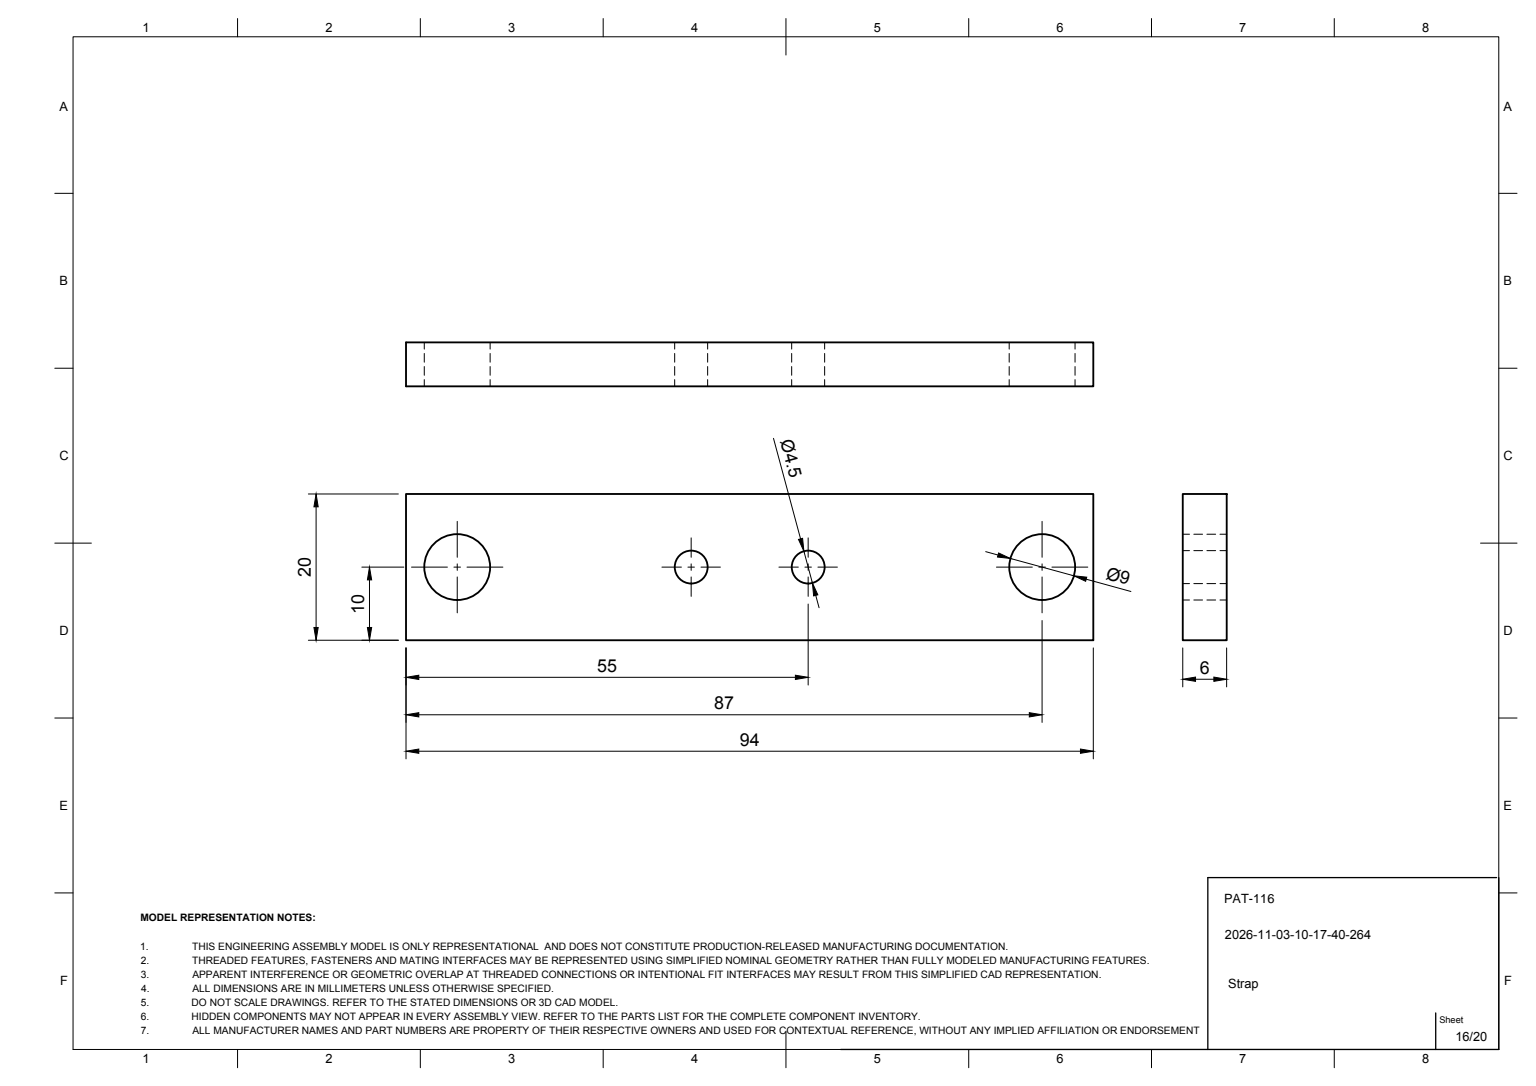
ISO-10303-21;
HEADER;
/* Generated by software containing ST-Developer
 * from STEP Tools, Inc. (www.steptools.com) 
 */

FILE_DESCRIPTION(
/* description */ ('V-block with clamp strap'),
/* implementation_level */ '2;1');

FILE_NAME(
/* name */ 'Strap.step',
/* time_stamp */ '2026-10-27T10:50:53-07:00',
/* author */ (''),
/* organization */ (''),
/* preprocessor_version */ 'ST-DEVELOPER v20.2',
/* originating_system */ 'Autodesk Translation Framework v15.17.0.0',
/* authorisation */ '');

FILE_SCHEMA (('AUTOMOTIVE_DESIGN { 1 0 10303 214 3 1 1 }'));
ENDSEC;

DATA;
#10=MECHANICAL_DESIGN_GEOMETRIC_PRESENTATION_REPRESENTATION('',(#279),#7344);
#237=SHAPE_REPRESENTATION_RELATIONSHIP('SRR','None',#7456,#258);
#258=ADVANCED_BREP_SHAPE_REPRESENTATION('',(#298),#7335);
#279=STYLED_ITEM('',(#7645),#298);
#298=MANIFOLD_SOLID_BREP('Body1',#4163);
#361=FACE_BOUND('',#1047,.T.);
#362=FACE_BOUND('',#1048,.T.);
#363=FACE_BOUND('',#1049,.T.);
#364=FACE_BOUND('',#1050,.T.);
#365=FACE_BOUND('',#1052,.T.);
#366=FACE_BOUND('',#1053,.T.);
#367=FACE_BOUND('',#1054,.T.);
#368=FACE_BOUND('',#1055,.T.);
#470=CIRCLE('',#4723,0.225);
#471=CIRCLE('',#4724,0.225);
#472=CIRCLE('',#4726,0.225);
#473=CIRCLE('',#4727,0.225);
#474=CIRCLE('',#4729,0.449999999999999);
#475=CIRCLE('',#4730,0.449999999999999);
#476=CIRCLE('',#4732,0.449999999999999);
#477=CIRCLE('',#4733,0.449999999999999);
#547=CYLINDRICAL_SURFACE('',#4722,0.225);
#548=CYLINDRICAL_SURFACE('',#4725,0.225);
#549=CYLINDRICAL_SURFACE('',#4728,0.449999999999999);
#550=CYLINDRICAL_SURFACE('',#4731,0.449999999999999);
#742=FACE_OUTER_BOUND('',#1038,.T.);
#743=FACE_OUTER_BOUND('',#1039,.T.);
#744=FACE_OUTER_BOUND('',#1040,.T.);
#745=FACE_OUTER_BOUND('',#1041,.T.);
#746=FACE_OUTER_BOUND('',#1042,.T.);
#747=FACE_OUTER_BOUND('',#1043,.T.);
#748=FACE_OUTER_BOUND('',#1044,.T.);
#749=FACE_OUTER_BOUND('',#1045,.T.);
#750=FACE_OUTER_BOUND('',#1046,.T.);
#751=FACE_OUTER_BOUND('',#1051,.T.);
#1038=EDGE_LOOP('',(#3516,#3517,#3518,#3519));
#1039=EDGE_LOOP('',(#3520,#3521,#3522,#3523));
#1040=EDGE_LOOP('',(#3524,#3525,#3526,#3527));
#1041=EDGE_LOOP('',(#3528,#3529,#3530,#3531));
#1042=EDGE_LOOP('',(#3532,#3533,#3534,#3535));
#1043=EDGE_LOOP('',(#3536,#3537,#3538,#3539));
#1044=EDGE_LOOP('',(#3540,#3541,#3542,#3543));
#1045=EDGE_LOOP('',(#3544,#3545,#3546,#3547));
#1046=EDGE_LOOP('',(#3548,#3549,#3550,#3551));
#1047=EDGE_LOOP('',(#3552));
#1048=EDGE_LOOP('',(#3553));
#1049=EDGE_LOOP('',(#3554));
#1050=EDGE_LOOP('',(#3555));
#1051=EDGE_LOOP('',(#3556,#3557,#3558,#3559));
#1052=EDGE_LOOP('',(#3560));
#1053=EDGE_LOOP('',(#3561));
#1054=EDGE_LOOP('',(#3562));
#1055=EDGE_LOOP('',(#3563));
#1413=LINE('',#7002,#1778);
#1414=LINE('',#7008,#1779);
#1415=LINE('',#7014,#1780);
#1416=LINE('',#7020,#1781);
#1417=LINE('',#7025,#1782);
#1418=LINE('',#7027,#1783);
#1419=LINE('',#7029,#1784);
#1420=LINE('',#7030,#1785);
#1421=LINE('',#7033,#1786);
#1422=LINE('',#7035,#1787);
#1423=LINE('',#7036,#1788);
#1424=LINE('',#7039,#1789);
#1425=LINE('',#7041,#1790);
#1426=LINE('',#7042,#1791);
#1427=LINE('',#7044,#1792);
#1428=LINE('',#7045,#1793);
#1778=VECTOR('',#5783,0.225);
#1779=VECTOR('',#5790,0.225);
#1780=VECTOR('',#5797,0.449999999999999);
#1781=VECTOR('',#5804,0.449999999999999);
#1782=VECTOR('',#5809,1.);
#1783=VECTOR('',#5810,1.);
#1784=VECTOR('',#5811,1.);
#1785=VECTOR('',#5812,1.);
#1786=VECTOR('',#5815,1.);
#1787=VECTOR('',#5816,1.);
#1788=VECTOR('',#5817,1.);
#1789=VECTOR('',#5820,1.);
#1790=VECTOR('',#5821,1.);
#1791=VECTOR('',#5822,1.);
#1792=VECTOR('',#5825,1.);
#1793=VECTOR('',#5826,1.);
#2101=VERTEX_POINT('',#6999);
#2102=VERTEX_POINT('',#7001);
#2103=VERTEX_POINT('',#7005);
#2104=VERTEX_POINT('',#7007);
#2105=VERTEX_POINT('',#7011);
#2106=VERTEX_POINT('',#7013);
#2107=VERTEX_POINT('',#7017);
#2108=VERTEX_POINT('',#7019);
#2109=VERTEX_POINT('',#7023);
#2110=VERTEX_POINT('',#7024);
#2111=VERTEX_POINT('',#7026);
#2112=VERTEX_POINT('',#7028);
#2113=VERTEX_POINT('',#7032);
#2114=VERTEX_POINT('',#7034);
#2115=VERTEX_POINT('',#7038);
#2116=VERTEX_POINT('',#7040);
#2584=EDGE_CURVE('',#2101,#2101,#470,.T.);
#2585=EDGE_CURVE('',#2101,#2102,#1413,.T.);
#2586=EDGE_CURVE('',#2102,#2102,#471,.T.);
#2587=EDGE_CURVE('',#2103,#2103,#472,.T.);
#2588=EDGE_CURVE('',#2103,#2104,#1414,.T.);
#2589=EDGE_CURVE('',#2104,#2104,#473,.T.);
#2590=EDGE_CURVE('',#2105,#2105,#474,.T.);
#2591=EDGE_CURVE('',#2105,#2106,#1415,.T.);
#2592=EDGE_CURVE('',#2106,#2106,#475,.T.);
#2593=EDGE_CURVE('',#2107,#2107,#476,.T.);
#2594=EDGE_CURVE('',#2107,#2108,#1416,.T.);
#2595=EDGE_CURVE('',#2108,#2108,#477,.T.);
#2596=EDGE_CURVE('',#2109,#2110,#1417,.T.);
#2597=EDGE_CURVE('',#2110,#2111,#1418,.T.);
#2598=EDGE_CURVE('',#2112,#2111,#1419,.T.);
#2599=EDGE_CURVE('',#2109,#2112,#1420,.T.);
#2600=EDGE_CURVE('',#2113,#2109,#1421,.T.);
#2601=EDGE_CURVE('',#2114,#2112,#1422,.T.);
#2602=EDGE_CURVE('',#2113,#2114,#1423,.T.);
#2603=EDGE_CURVE('',#2115,#2113,#1424,.T.);
#2604=EDGE_CURVE('',#2116,#2114,#1425,.T.);
#2605=EDGE_CURVE('',#2115,#2116,#1426,.T.);
#2606=EDGE_CURVE('',#2110,#2115,#1427,.T.);
#2607=EDGE_CURVE('',#2111,#2116,#1428,.T.);
#3516=ORIENTED_EDGE('',*,*,#2584,.F.);
#3517=ORIENTED_EDGE('',*,*,#2585,.T.);
#3518=ORIENTED_EDGE('',*,*,#2586,.F.);
#3519=ORIENTED_EDGE('',*,*,#2585,.F.);
#3520=ORIENTED_EDGE('',*,*,#2587,.F.);
#3521=ORIENTED_EDGE('',*,*,#2588,.T.);
#3522=ORIENTED_EDGE('',*,*,#2589,.F.);
#3523=ORIENTED_EDGE('',*,*,#2588,.F.);
#3524=ORIENTED_EDGE('',*,*,#2590,.F.);
#3525=ORIENTED_EDGE('',*,*,#2591,.T.);
#3526=ORIENTED_EDGE('',*,*,#2592,.F.);
#3527=ORIENTED_EDGE('',*,*,#2591,.F.);
#3528=ORIENTED_EDGE('',*,*,#2593,.F.);
#3529=ORIENTED_EDGE('',*,*,#2594,.T.);
#3530=ORIENTED_EDGE('',*,*,#2595,.F.);
#3531=ORIENTED_EDGE('',*,*,#2594,.F.);
#3532=ORIENTED_EDGE('',*,*,#2596,.T.);
#3533=ORIENTED_EDGE('',*,*,#2597,.T.);
#3534=ORIENTED_EDGE('',*,*,#2598,.F.);
#3535=ORIENTED_EDGE('',*,*,#2599,.F.);
#3536=ORIENTED_EDGE('',*,*,#2600,.T.);
#3537=ORIENTED_EDGE('',*,*,#2599,.T.);
#3538=ORIENTED_EDGE('',*,*,#2601,.F.);
#3539=ORIENTED_EDGE('',*,*,#2602,.F.);
#3540=ORIENTED_EDGE('',*,*,#2603,.T.);
#3541=ORIENTED_EDGE('',*,*,#2602,.T.);
#3542=ORIENTED_EDGE('',*,*,#2604,.F.);
#3543=ORIENTED_EDGE('',*,*,#2605,.F.);
#3544=ORIENTED_EDGE('',*,*,#2606,.T.);
#3545=ORIENTED_EDGE('',*,*,#2605,.T.);
#3546=ORIENTED_EDGE('',*,*,#2607,.F.);
#3547=ORIENTED_EDGE('',*,*,#2597,.F.);
#3548=ORIENTED_EDGE('',*,*,#2607,.T.);
#3549=ORIENTED_EDGE('',*,*,#2604,.T.);
#3550=ORIENTED_EDGE('',*,*,#2601,.T.);
#3551=ORIENTED_EDGE('',*,*,#2598,.T.);
#3552=ORIENTED_EDGE('',*,*,#2586,.T.);
#3553=ORIENTED_EDGE('',*,*,#2589,.T.);
#3554=ORIENTED_EDGE('',*,*,#2592,.T.);
#3555=ORIENTED_EDGE('',*,*,#2595,.T.);
#3556=ORIENTED_EDGE('',*,*,#2606,.F.);
#3557=ORIENTED_EDGE('',*,*,#2596,.F.);
#3558=ORIENTED_EDGE('',*,*,#2600,.F.);
#3559=ORIENTED_EDGE('',*,*,#2603,.F.);
#3560=ORIENTED_EDGE('',*,*,#2584,.T.);
#3561=ORIENTED_EDGE('',*,*,#2587,.T.);
#3562=ORIENTED_EDGE('',*,*,#2590,.T.);
#3563=ORIENTED_EDGE('',*,*,#2593,.T.);
#3868=PLANE('',#4734);
#3869=PLANE('',#4735);
#3870=PLANE('',#4736);
#3871=PLANE('',#4737);
#3872=PLANE('',#4738);
#3873=PLANE('',#4739);
#4088=ADVANCED_FACE('',(#742),#547,.F.);
#4089=ADVANCED_FACE('',(#743),#548,.F.);
#4090=ADVANCED_FACE('',(#744),#549,.F.);
#4091=ADVANCED_FACE('',(#745),#550,.F.);
#4092=ADVANCED_FACE('',(#746),#3868,.T.);
#4093=ADVANCED_FACE('',(#747),#3869,.T.);
#4094=ADVANCED_FACE('',(#748),#3870,.T.);
#4095=ADVANCED_FACE('',(#749),#3871,.T.);
#4096=ADVANCED_FACE('',(#750,#361,#362,#363,#364),#3872,.T.);
#4097=ADVANCED_FACE('',(#751,#365,#366,#367,#368),#3873,.F.);
#4163=CLOSED_SHELL('',(#4088,#4089,#4090,#4091,#4092,#4093,#4094,#4095,
#4096,#4097));
#4721=AXIS2_PLACEMENT_3D('',#6997,#5777,#5778);
#4722=AXIS2_PLACEMENT_3D('',#6998,#5779,#5780);
#4723=AXIS2_PLACEMENT_3D('',#7000,#5781,#5782);
#4724=AXIS2_PLACEMENT_3D('',#7003,#5784,#5785);
#4725=AXIS2_PLACEMENT_3D('',#7004,#5786,#5787);
#4726=AXIS2_PLACEMENT_3D('',#7006,#5788,#5789);
#4727=AXIS2_PLACEMENT_3D('',#7009,#5791,#5792);
#4728=AXIS2_PLACEMENT_3D('',#7010,#5793,#5794);
#4729=AXIS2_PLACEMENT_3D('',#7012,#5795,#5796);
#4730=AXIS2_PLACEMENT_3D('',#7015,#5798,#5799);
#4731=AXIS2_PLACEMENT_3D('',#7016,#5800,#5801);
#4732=AXIS2_PLACEMENT_3D('',#7018,#5802,#5803);
#4733=AXIS2_PLACEMENT_3D('',#7021,#5805,#5806);
#4734=AXIS2_PLACEMENT_3D('',#7022,#5807,#5808);
#4735=AXIS2_PLACEMENT_3D('',#7031,#5813,#5814);
#4736=AXIS2_PLACEMENT_3D('',#7037,#5818,#5819);
#4737=AXIS2_PLACEMENT_3D('',#7043,#5823,#5824);
#4738=AXIS2_PLACEMENT_3D('',#7046,#5827,#5828);
#4739=AXIS2_PLACEMENT_3D('',#7047,#5829,#5830);
#5777=DIRECTION('axis',(0.,0.,1.));
#5778=DIRECTION('refdir',(1.,0.,0.));
#5779=DIRECTION('center_axis',(0.,0.,1.));
#5780=DIRECTION('ref_axis',(1.,0.,0.));
#5781=DIRECTION('center_axis',(0.,0.,1.));
#5782=DIRECTION('ref_axis',(1.,0.,0.));
#5783=DIRECTION('',(0.,0.,1.));
#5784=DIRECTION('center_axis',(0.,0.,-1.));
#5785=DIRECTION('ref_axis',(1.,0.,0.));
#5786=DIRECTION('center_axis',(0.,0.,1.));
#5787=DIRECTION('ref_axis',(1.,0.,0.));
#5788=DIRECTION('center_axis',(0.,0.,1.));
#5789=DIRECTION('ref_axis',(1.,0.,0.));
#5790=DIRECTION('',(0.,0.,1.));
#5791=DIRECTION('center_axis',(0.,0.,-1.));
#5792=DIRECTION('ref_axis',(1.,0.,0.));
#5793=DIRECTION('center_axis',(0.,0.,1.));
#5794=DIRECTION('ref_axis',(1.,0.,0.));
#5795=DIRECTION('center_axis',(0.,0.,1.));
#5796=DIRECTION('ref_axis',(1.,0.,0.));
#5797=DIRECTION('',(0.,0.,1.));
#5798=DIRECTION('center_axis',(0.,0.,-1.));
#5799=DIRECTION('ref_axis',(1.,0.,0.));
#5800=DIRECTION('center_axis',(0.,0.,1.));
#5801=DIRECTION('ref_axis',(1.,0.,0.));
#5802=DIRECTION('center_axis',(0.,0.,1.));
#5803=DIRECTION('ref_axis',(1.,0.,0.));
#5804=DIRECTION('',(0.,0.,1.));
#5805=DIRECTION('center_axis',(0.,0.,-1.));
#5806=DIRECTION('ref_axis',(1.,0.,0.));
#5807=DIRECTION('center_axis',(0.,1.,0.));
#5808=DIRECTION('ref_axis',(-1.,0.,0.));
#5809=DIRECTION('',(-1.,0.,0.));
#5810=DIRECTION('',(0.,0.,1.));
#5811=DIRECTION('',(-1.,0.,0.));
#5812=DIRECTION('',(0.,0.,1.));
#5813=DIRECTION('center_axis',(1.,0.,0.));
#5814=DIRECTION('ref_axis',(0.,1.,0.));
#5815=DIRECTION('',(0.,1.,0.));
#5816=DIRECTION('',(0.,1.,0.));
#5817=DIRECTION('',(0.,0.,1.));
#5818=DIRECTION('center_axis',(0.,-1.,0.));
#5819=DIRECTION('ref_axis',(1.,0.,0.));
#5820=DIRECTION('',(1.,0.,0.));
#5821=DIRECTION('',(1.,0.,0.));
#5822=DIRECTION('',(0.,0.,1.));
#5823=DIRECTION('center_axis',(-1.,0.,0.));
#5824=DIRECTION('ref_axis',(0.,-1.,0.));
#5825=DIRECTION('',(0.,-1.,0.));
#5826=DIRECTION('',(0.,-1.,0.));
#5827=DIRECTION('center_axis',(0.,0.,1.));
#5828=DIRECTION('ref_axis',(1.,0.,0.));
#5829=DIRECTION('center_axis',(0.,0.,1.));
#5830=DIRECTION('ref_axis',(1.,0.,0.));
#6997=CARTESIAN_POINT('',(0.,0.,0.));
#6998=CARTESIAN_POINT('Origin',(10.,-0.8,6.42132034));
#6999=CARTESIAN_POINT('',(9.775,-0.8,6.52132034));
#7000=CARTESIAN_POINT('Origin',(10.,-0.8,6.52132034));
#7001=CARTESIAN_POINT('',(9.775,-0.8,7.12132034));
#7002=CARTESIAN_POINT('',(9.775,-0.8,6.42132034));
#7003=CARTESIAN_POINT('Origin',(10.,-0.8,7.12132034));
#7004=CARTESIAN_POINT('Origin',(10.,0.8,6.42132034));
#7005=CARTESIAN_POINT('',(9.775,0.8,6.52132034));
#7006=CARTESIAN_POINT('Origin',(10.,0.8,6.52132034));
#7007=CARTESIAN_POINT('',(9.775,0.8,7.12132034));
#7008=CARTESIAN_POINT('',(9.775,0.8,6.42132034));
#7009=CARTESIAN_POINT('Origin',(10.,0.8,7.12132034));
#7010=CARTESIAN_POINT('Origin',(10.,-4.,6.42132034));
#7011=CARTESIAN_POINT('',(9.55,-4.,6.52132034));
#7012=CARTESIAN_POINT('Origin',(10.,-4.,6.52132034));
#7013=CARTESIAN_POINT('',(9.55,-4.,7.12132034));
#7014=CARTESIAN_POINT('',(9.55,-4.,6.42132034));
#7015=CARTESIAN_POINT('Origin',(10.,-4.,7.12132034));
#7016=CARTESIAN_POINT('Origin',(10.,4.,6.42132034));
#7017=CARTESIAN_POINT('',(9.55,4.,6.52132034));
#7018=CARTESIAN_POINT('Origin',(10.,4.,6.52132034));
#7019=CARTESIAN_POINT('',(9.55,4.,7.12132034));
#7020=CARTESIAN_POINT('',(9.55,4.,6.42132034));
#7021=CARTESIAN_POINT('Origin',(10.,4.,7.12132034));
#7022=CARTESIAN_POINT('Origin',(11.,4.7,6.52132034));
#7023=CARTESIAN_POINT('',(11.,4.7,6.52132034));
#7024=CARTESIAN_POINT('',(9.,4.7,6.52132034));
#7025=CARTESIAN_POINT('',(11.,4.7,6.52132034));
#7026=CARTESIAN_POINT('',(9.,4.7,7.12132034));
#7027=CARTESIAN_POINT('',(9.,4.7,6.52132034));
#7028=CARTESIAN_POINT('',(11.,4.7,7.12132034));
#7029=CARTESIAN_POINT('',(11.,4.7,7.12132034));
#7030=CARTESIAN_POINT('',(11.,4.7,6.52132034));
#7031=CARTESIAN_POINT('Origin',(11.,-4.7,6.52132034));
#7032=CARTESIAN_POINT('',(11.,-4.7,6.52132034));
#7033=CARTESIAN_POINT('',(11.,-4.7,6.52132034));
#7034=CARTESIAN_POINT('',(11.,-4.7,7.12132034));
#7035=CARTESIAN_POINT('',(11.,-4.7,7.12132034));
#7036=CARTESIAN_POINT('',(11.,-4.7,6.52132034));
#7037=CARTESIAN_POINT('Origin',(9.,-4.7,6.52132034));
#7038=CARTESIAN_POINT('',(9.,-4.7,6.52132034));
#7039=CARTESIAN_POINT('',(9.,-4.7,6.52132034));
#7040=CARTESIAN_POINT('',(9.,-4.7,7.12132034));
#7041=CARTESIAN_POINT('',(9.,-4.7,7.12132034));
#7042=CARTESIAN_POINT('',(9.,-4.7,6.52132034));
#7043=CARTESIAN_POINT('Origin',(9.,4.7,6.52132034));
#7044=CARTESIAN_POINT('',(9.,4.7,6.52132034));
#7045=CARTESIAN_POINT('',(9.,4.7,7.12132034));
#7046=CARTESIAN_POINT('Origin',(10.,0.,7.12132034));
#7047=CARTESIAN_POINT('Origin',(10.,0.,6.52132034));
#7309=UNCERTAINTY_MEASURE_WITH_UNIT(LENGTH_MEASURE(0.001),#7345,
'DISTANCE_ACCURACY_VALUE',
'Maximum model space distance between geometric entities at asserted c
onnectivities');
#7318=UNCERTAINTY_MEASURE_WITH_UNIT(LENGTH_MEASURE(0.001),#7345,
'DISTANCE_ACCURACY_VALUE',
'Maximum model space distance between geometric entities at asserted c
onnectivities');
#7335=(
GEOMETRIC_REPRESENTATION_CONTEXT(3)
GLOBAL_UNCERTAINTY_ASSIGNED_CONTEXT((#7309))
GLOBAL_UNIT_ASSIGNED_CONTEXT((#7345,#7347,#7348))
REPRESENTATION_CONTEXT('','3D')
);
#7344=(
GEOMETRIC_REPRESENTATION_CONTEXT(3)
GLOBAL_UNCERTAINTY_ASSIGNED_CONTEXT((#7318))
GLOBAL_UNIT_ASSIGNED_CONTEXT((#7345,#7347,#7348))
REPRESENTATION_CONTEXT('','3D')
);
#7345=(
LENGTH_UNIT()
NAMED_UNIT(*)
SI_UNIT(.CENTI.,.METRE.)
);
#7347=(
NAMED_UNIT(*)
PLANE_ANGLE_UNIT()
SI_UNIT($,.RADIAN.)
);
#7348=(
NAMED_UNIT(*)
SI_UNIT($,.STERADIAN.)
SOLID_ANGLE_UNIT()
);
#7365=SHAPE_DEFINITION_REPRESENTATION(#7413,#7456);
#7413=PRODUCT_DEFINITION_SHAPE('',$,#7482);
#7456=SHAPE_REPRESENTATION('',(#4721),#7335);
#7465=PRODUCT_DEFINITION_CONTEXT('part definition',#7542,'design');
#7482=PRODUCT_DEFINITION('Strap','Strap',#7507,#7465);
#7507=PRODUCT_DEFINITION_FORMATION('',$,#7560);
#7542=APPLICATION_CONTEXT(
'Core Data for Automotive Mechanical Design Process');
#7543=PRODUCT_CONTEXT('part definition',#7542,'mechanical');
#7560=PRODUCT('Strap','Strap','Strap',(#7543));
#7639=COLOUR_RGB('Off White',0.89,0.88,0.83);
#7640=FILL_AREA_STYLE_COLOUR('',#7639);
#7641=FILL_AREA_STYLE('',(#7640));
#7642=SURFACE_STYLE_FILL_AREA(#7641);
#7643=SURFACE_SIDE_STYLE('',(#7642));
#7644=SURFACE_STYLE_USAGE(.BOTH.,#7643);
#7645=PRESENTATION_STYLE_ASSIGNMENT((#7644));
ENDSEC;
END-ISO-10303-21;
